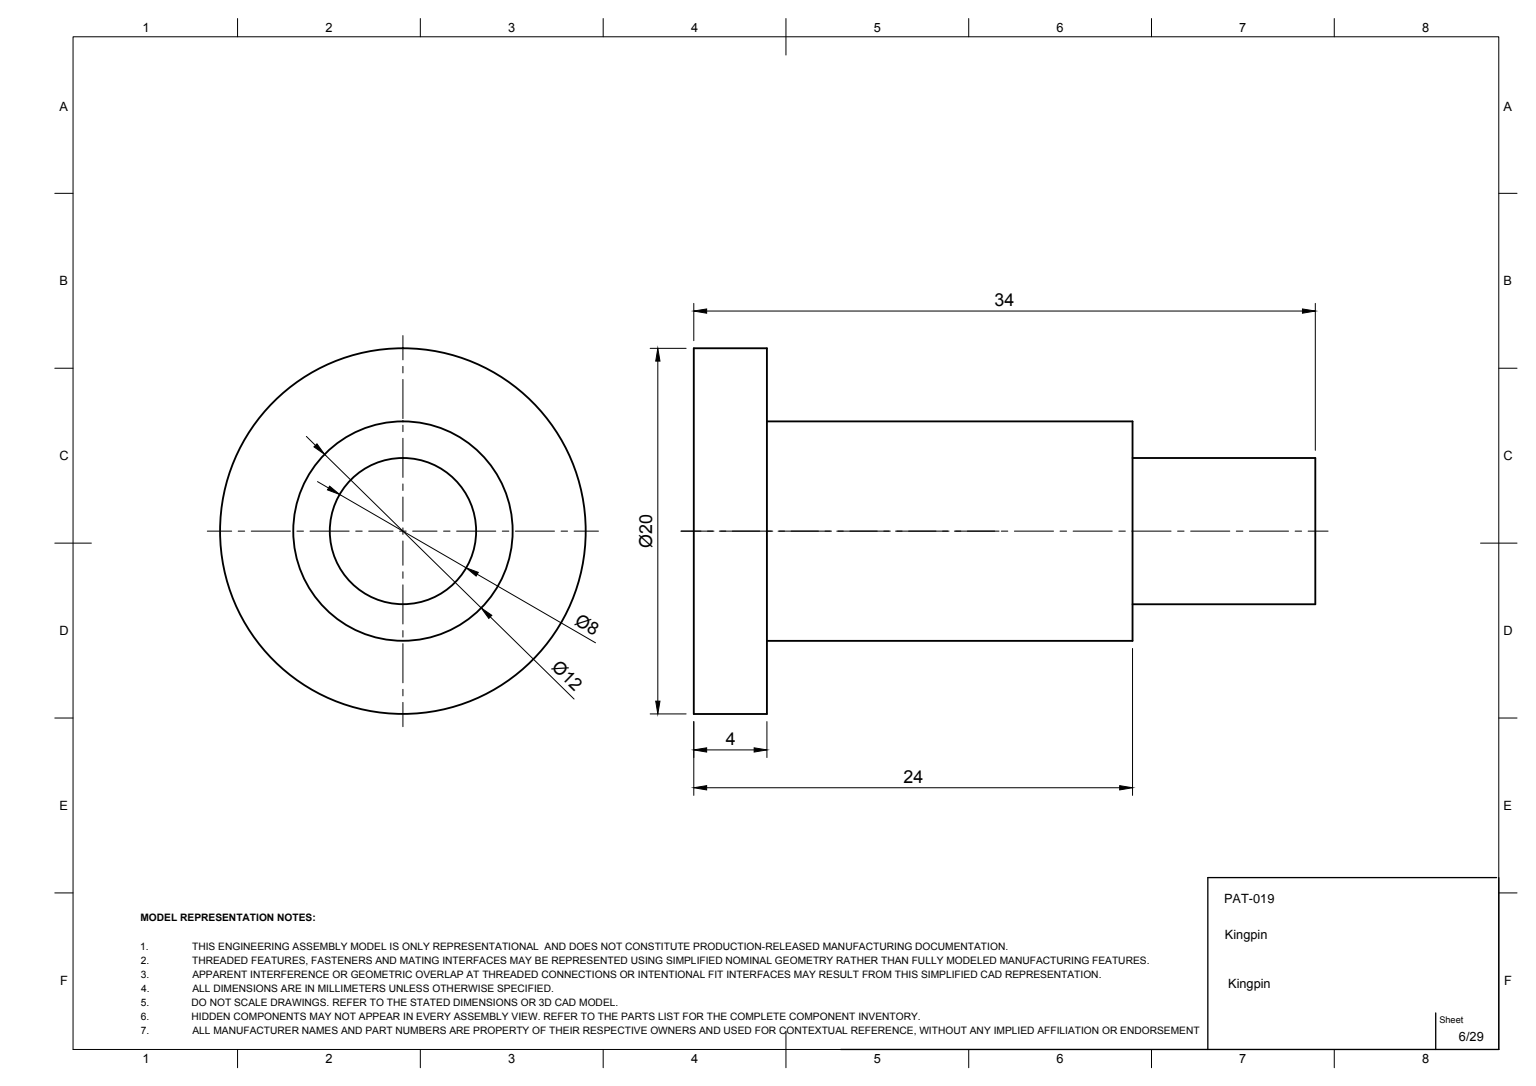
ISO-10303-21;
HEADER;
/* Generated by software containing ST-Developer
 * from STEP Tools, Inc. (www.steptools.com) 
 */

FILE_DESCRIPTION(
/* description */ ('Caster wheel assembly'),
/* implementation_level */ '2;1');

FILE_NAME(
/* name */ 'Kingpin.step',
/* time_stamp */ '2026-10-28T03:23:56-07:00',
/* author */ (''),
/* organization */ (''),
/* preprocessor_version */ 'ST-DEVELOPER v20.2',
/* originating_system */ 'Autodesk Translation Framework v15.17.0.0',
/* authorisation */ '');

FILE_SCHEMA (('AUTOMOTIVE_DESIGN { 1 0 10303 214 3 1 1 }'));
ENDSEC;

DATA;
#10=MECHANICAL_DESIGN_GEOMETRIC_PRESENTATION_REPRESENTATION('',(#223),#5385);
#179=SHAPE_REPRESENTATION_RELATIONSHIP('SRR','None',#5474,#201);
#201=ADVANCED_BREP_SHAPE_REPRESENTATION('',(#253),#5361);
#223=STYLED_ITEM('',(#5672),#253);
#253=MANIFOLD_SOLID_BREP('Body1',#2650);
#291=FACE_BOUND('',#613,.T.);
#292=FACE_BOUND('',#618,.T.);
#339=PLANE('',#2951);
#340=PLANE('',#2952);
#341=PLANE('',#2957);
#342=PLANE('',#2960);
#432=FACE_OUTER_BOUND('',#610,.T.);
#433=FACE_OUTER_BOUND('',#611,.T.);
#434=FACE_OUTER_BOUND('',#612,.T.);
#435=FACE_OUTER_BOUND('',#614,.T.);
#436=FACE_OUTER_BOUND('',#615,.T.);
#437=FACE_OUTER_BOUND('',#616,.T.);
#438=FACE_OUTER_BOUND('',#617,.T.);
#610=EDGE_LOOP('',(#1836,#1837,#1838,#1839));
#611=EDGE_LOOP('',(#1840));
#612=EDGE_LOOP('',(#1841));
#613=EDGE_LOOP('',(#1842));
#614=EDGE_LOOP('',(#1843,#1844,#1845,#1846));
#615=EDGE_LOOP('',(#1847));
#616=EDGE_LOOP('',(#1848,#1849,#1850,#1851));
#617=EDGE_LOOP('',(#1852));
#618=EDGE_LOOP('',(#1853));
#826=LINE('',#4264,#960);
#827=LINE('',#4275,#961);
#828=LINE('',#4279,#962);
#960=VECTOR('',#3375,0.4);
#961=VECTOR('',#3390,1.);
#962=VECTOR('',#3395,0.6);
#1087=CIRCLE('',#2949,0.4);
#1088=CIRCLE('',#2950,0.4);
#1089=CIRCLE('',#2953,1.);
#1090=CIRCLE('',#2954,0.6);
#1091=CIRCLE('',#2956,1.);
#1092=CIRCLE('',#2959,0.6);
#1254=VERTEX_POINT('',#4261);
#1255=VERTEX_POINT('',#4263);
#1256=VERTEX_POINT('',#4268);
#1257=VERTEX_POINT('',#4270);
#1258=VERTEX_POINT('',#4273);
#1259=VERTEX_POINT('',#4278);
#1486=EDGE_CURVE('',#1254,#1254,#1087,.T.);
#1487=EDGE_CURVE('',#1254,#1255,#826,.T.);
#1488=EDGE_CURVE('',#1255,#1255,#1088,.T.);
#1489=EDGE_CURVE('',#1256,#1256,#1089,.T.);
#1490=EDGE_CURVE('',#1257,#1257,#1090,.T.);
#1491=EDGE_CURVE('',#1258,#1258,#1091,.T.);
#1492=EDGE_CURVE('',#1258,#1256,#827,.T.);
#1493=EDGE_CURVE('',#1257,#1259,#828,.T.);
#1494=EDGE_CURVE('',#1259,#1259,#1092,.T.);
#1836=ORIENTED_EDGE('',*,*,#1486,.F.);
#1837=ORIENTED_EDGE('',*,*,#1487,.T.);
#1838=ORIENTED_EDGE('',*,*,#1488,.T.);
#1839=ORIENTED_EDGE('',*,*,#1487,.F.);
#1840=ORIENTED_EDGE('',*,*,#1488,.F.);
#1841=ORIENTED_EDGE('',*,*,#1489,.F.);
#1842=ORIENTED_EDGE('',*,*,#1490,.T.);
#1843=ORIENTED_EDGE('',*,*,#1491,.F.);
#1844=ORIENTED_EDGE('',*,*,#1492,.T.);
#1845=ORIENTED_EDGE('',*,*,#1489,.T.);
#1846=ORIENTED_EDGE('',*,*,#1492,.F.);
#1847=ORIENTED_EDGE('',*,*,#1491,.T.);
#1848=ORIENTED_EDGE('',*,*,#1490,.F.);
#1849=ORIENTED_EDGE('',*,*,#1493,.T.);
#1850=ORIENTED_EDGE('',*,*,#1494,.T.);
#1851=ORIENTED_EDGE('',*,*,#1493,.F.);
#1852=ORIENTED_EDGE('',*,*,#1494,.F.);
#1853=ORIENTED_EDGE('',*,*,#1486,.T.);
#2433=CYLINDRICAL_SURFACE('',#2948,0.4);
#2434=CYLINDRICAL_SURFACE('',#2955,1.);
#2435=CYLINDRICAL_SURFACE('',#2958,0.6);
#2492=ADVANCED_FACE('',(#432),#2433,.T.);
#2493=ADVANCED_FACE('',(#433),#339,.F.);
#2494=ADVANCED_FACE('',(#434,#291),#340,.F.);
#2495=ADVANCED_FACE('',(#435),#2434,.T.);
#2496=ADVANCED_FACE('',(#436),#341,.T.);
#2497=ADVANCED_FACE('',(#437),#2435,.T.);
#2498=ADVANCED_FACE('',(#438,#292),#342,.F.);
#2650=CLOSED_SHELL('',(#2492,#2493,#2494,#2495,#2496,#2497,#2498));
#2947=AXIS2_PLACEMENT_3D('',#4259,#3369,#3370);
#2948=AXIS2_PLACEMENT_3D('',#4260,#3371,#3372);
#2949=AXIS2_PLACEMENT_3D('',#4262,#3373,#3374);
#2950=AXIS2_PLACEMENT_3D('',#4265,#3376,#3377);
#2951=AXIS2_PLACEMENT_3D('',#4266,#3378,#3379);
#2952=AXIS2_PLACEMENT_3D('',#4267,#3380,#3381);
#2953=AXIS2_PLACEMENT_3D('',#4269,#3382,#3383);
#2954=AXIS2_PLACEMENT_3D('',#4271,#3384,#3385);
#2955=AXIS2_PLACEMENT_3D('',#4272,#3386,#3387);
#2956=AXIS2_PLACEMENT_3D('',#4274,#3388,#3389);
#2957=AXIS2_PLACEMENT_3D('',#4276,#3391,#3392);
#2958=AXIS2_PLACEMENT_3D('',#4277,#3393,#3394);
#2959=AXIS2_PLACEMENT_3D('',#4280,#3396,#3397);
#2960=AXIS2_PLACEMENT_3D('',#4281,#3398,#3399);
#3369=DIRECTION('axis',(0.,0.,1.));
#3370=DIRECTION('refdir',(1.,0.,0.));
#3371=DIRECTION('center_axis',(0.,0.,1.));
#3372=DIRECTION('ref_axis',(1.,0.,0.));
#3373=DIRECTION('center_axis',(0.,0.,1.));
#3374=DIRECTION('ref_axis',(1.,0.,0.));
#3375=DIRECTION('',(0.,0.,-1.));
#3376=DIRECTION('center_axis',(0.,0.,1.));
#3377=DIRECTION('ref_axis',(1.,0.,0.));
#3378=DIRECTION('center_axis',(0.,0.,1.));
#3379=DIRECTION('ref_axis',(1.,0.,0.));
#3380=DIRECTION('center_axis',(0.,0.,1.));
#3381=DIRECTION('ref_axis',(1.,0.,0.));
#3382=DIRECTION('center_axis',(0.,0.,1.));
#3383=DIRECTION('ref_axis',(1.,0.,0.));
#3384=DIRECTION('center_axis',(0.,0.,1.));
#3385=DIRECTION('ref_axis',(1.,0.,0.));
#3386=DIRECTION('center_axis',(0.,0.,1.));
#3387=DIRECTION('ref_axis',(1.,0.,0.));
#3388=DIRECTION('center_axis',(0.,0.,1.));
#3389=DIRECTION('ref_axis',(1.,0.,0.));
#3390=DIRECTION('',(0.,0.,-1.));
#3391=DIRECTION('center_axis',(0.,0.,1.));
#3392=DIRECTION('ref_axis',(1.,0.,0.));
#3393=DIRECTION('center_axis',(0.,0.,1.));
#3394=DIRECTION('ref_axis',(1.,0.,0.));
#3395=DIRECTION('',(0.,0.,-1.));
#3396=DIRECTION('center_axis',(0.,0.,1.));
#3397=DIRECTION('ref_axis',(1.,0.,0.));
#3398=DIRECTION('center_axis',(0.,0.,1.));
#3399=DIRECTION('ref_axis',(1.,0.,0.));
#4259=CARTESIAN_POINT('',(0.,0.,0.));
#4260=CARTESIAN_POINT('Origin',(-2.,0.,7.5));
#4261=CARTESIAN_POINT('',(-2.4,-4.89858719658941E-17,8.5));
#4262=CARTESIAN_POINT('Origin',(-2.,0.,8.5));
#4263=CARTESIAN_POINT('',(-2.4,-4.89858719658941E-17,7.5));
#4264=CARTESIAN_POINT('',(-2.4,-4.89858719658941E-17,7.5));
#4265=CARTESIAN_POINT('Origin',(-2.,0.,7.5));
#4266=CARTESIAN_POINT('Origin',(-2.,0.,7.5));
#4267=CARTESIAN_POINT('Origin',(-2.,0.,10.5));
#4268=CARTESIAN_POINT('',(-3.,-1.22464679914735E-16,10.5));
#4269=CARTESIAN_POINT('Origin',(-2.,0.,10.5));
#4270=CARTESIAN_POINT('',(-2.6,-7.34788079488412E-17,10.5));
#4271=CARTESIAN_POINT('Origin',(-2.,0.,10.5));
#4272=CARTESIAN_POINT('Origin',(-2.,0.,10.5));
#4273=CARTESIAN_POINT('',(-3.,-1.22464679914735E-16,10.9));
#4274=CARTESIAN_POINT('Origin',(-2.,0.,10.9));
#4275=CARTESIAN_POINT('',(-3.,-1.22464679914735E-16,10.5));
#4276=CARTESIAN_POINT('Origin',(-2.,0.,10.9));
#4277=CARTESIAN_POINT('Origin',(-2.,0.,8.5));
#4278=CARTESIAN_POINT('',(-2.6,-7.34788079488412E-17,8.5));
#4279=CARTESIAN_POINT('',(-2.6,-7.34788079488412E-17,8.5));
#4280=CARTESIAN_POINT('Origin',(-2.,0.,8.5));
#4281=CARTESIAN_POINT('Origin',(-2.,0.,8.5));
#5333=UNCERTAINTY_MEASURE_WITH_UNIT(LENGTH_MEASURE(0.001),#5386,
'DISTANCE_ACCURACY_VALUE',
'Maximum model space distance between geometric entities at asserted c
onnectivities');
#5357=UNCERTAINTY_MEASURE_WITH_UNIT(LENGTH_MEASURE(0.001),#5386,
'DISTANCE_ACCURACY_VALUE',
'Maximum model space distance between geometric entities at asserted c
onnectivities');
#5361=(
GEOMETRIC_REPRESENTATION_CONTEXT(3)
GLOBAL_UNCERTAINTY_ASSIGNED_CONTEXT((#5333))
GLOBAL_UNIT_ASSIGNED_CONTEXT((#5386,#5388,#5389))
REPRESENTATION_CONTEXT('','3D')
);
#5385=(
GEOMETRIC_REPRESENTATION_CONTEXT(3)
GLOBAL_UNCERTAINTY_ASSIGNED_CONTEXT((#5357))
GLOBAL_UNIT_ASSIGNED_CONTEXT((#5386,#5388,#5389))
REPRESENTATION_CONTEXT('','3D')
);
#5386=(
LENGTH_UNIT()
NAMED_UNIT(*)
SI_UNIT(.CENTI.,.METRE.)
);
#5388=(
NAMED_UNIT(*)
PLANE_ANGLE_UNIT()
SI_UNIT($,.RADIAN.)
);
#5389=(
NAMED_UNIT(*)
SI_UNIT($,.STERADIAN.)
SOLID_ANGLE_UNIT()
);
#5393=SHAPE_DEFINITION_REPRESENTATION(#5420,#5474);
#5420=PRODUCT_DEFINITION_SHAPE('',$,#5502);
#5474=SHAPE_REPRESENTATION('',(#2947),#5361);
#5498=PRODUCT_DEFINITION_CONTEXT('part definition',#5581,'design');
#5502=PRODUCT_DEFINITION('Kingpin','Kingpin',#5529,#5498);
#5529=PRODUCT_DEFINITION_FORMATION('',$,#5586);
#5581=APPLICATION_CONTEXT(
'Core Data for Automotive Mechanical Design Process');
#5582=PRODUCT_CONTEXT('part definition',#5581,'mechanical');
#5586=PRODUCT('Kingpin','Kingpin','Kingpin',(#5582));
#5666=COLOUR_RGB('Grey',0.48,0.52,0.57);
#5667=FILL_AREA_STYLE_COLOUR('',#5666);
#5668=FILL_AREA_STYLE('',(#5667));
#5669=SURFACE_STYLE_FILL_AREA(#5668);
#5670=SURFACE_SIDE_STYLE('',(#5669));
#5671=SURFACE_STYLE_USAGE(.BOTH.,#5670);
#5672=PRESENTATION_STYLE_ASSIGNMENT((#5671));
ENDSEC;
END-ISO-10303-21;
